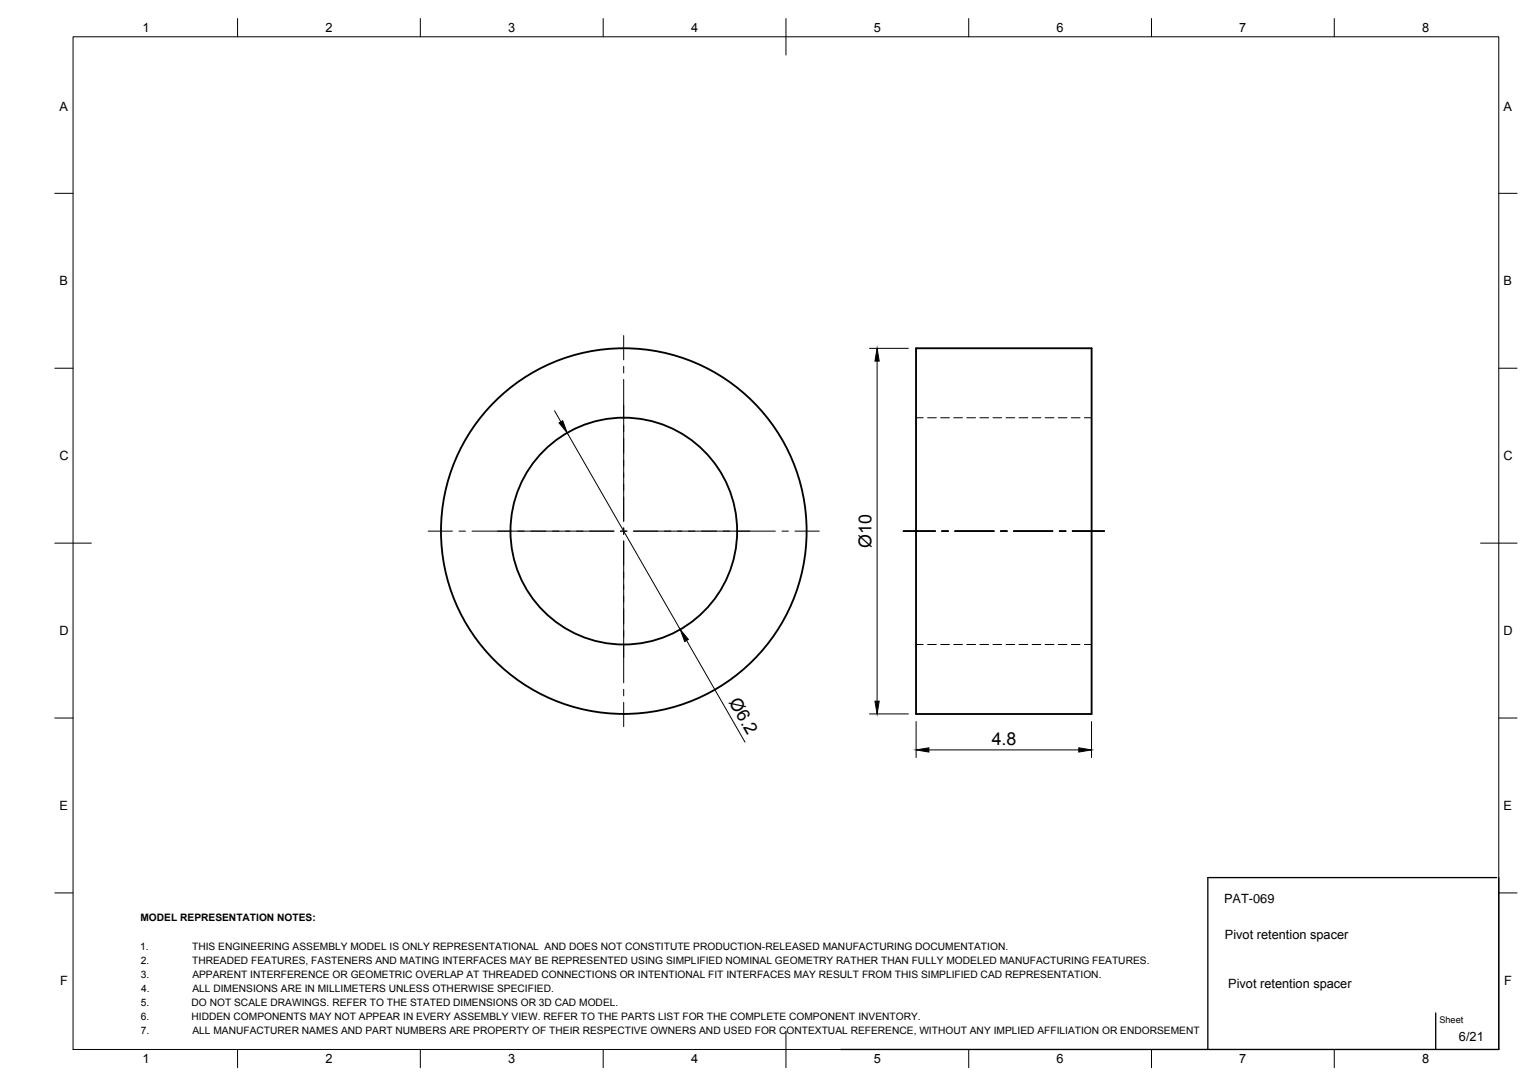
ISO-10303-21;
HEADER;
/* Generated by software containing ST-Developer
 * from STEP Tools, Inc. (www.steptools.com) 
 */

FILE_DESCRIPTION(
/* description */ ('Located fixture plate with toggle clamp'),
/* implementation_level */ '2;1');

FILE_NAME(
/* name */ 'Pivot retention spacer.step',
/* time_stamp */ '2026-10-27T21:36:12-07:00',
/* author */ (''),
/* organization */ (''),
/* preprocessor_version */ 'ST-DEVELOPER v20.2',
/* originating_system */ 'Autodesk Translation Framework v15.17.0.0',
/* authorisation */ '');

FILE_SCHEMA (('AUTOMOTIVE_DESIGN { 1 0 10303 214 3 1 1 }'));
ENDSEC;

DATA;
#10=MECHANICAL_DESIGN_GEOMETRIC_PRESENTATION_REPRESENTATION('',(#343),#9285);
#295=SHAPE_REPRESENTATION_RELATIONSHIP('SRR','None',#9421,#319);
#319=ADVANCED_BREP_SHAPE_REPRESENTATION('',(#364),#9283);
#343=STYLED_ITEM('',(#9626),#364);
#364=MANIFOLD_SOLID_BREP('Body1',#5194);
#483=FACE_BOUND('',#1374,.T.);
#484=FACE_BOUND('',#1376,.T.);
#668=PLANE('',#5971);
#669=PLANE('',#5972);
#959=FACE_OUTER_BOUND('',#1371,.T.);
#960=FACE_OUTER_BOUND('',#1372,.T.);
#961=FACE_OUTER_BOUND('',#1373,.T.);
#962=FACE_OUTER_BOUND('',#1375,.T.);
#1371=EDGE_LOOP('',(#4756,#4757,#4758,#4759));
#1372=EDGE_LOOP('',(#4760,#4761,#4762,#4763));
#1373=EDGE_LOOP('',(#4764));
#1374=EDGE_LOOP('',(#4765));
#1375=EDGE_LOOP('',(#4766));
#1376=EDGE_LOOP('',(#4767));
#1572=CIRCLE('',#5966,0.31);
#1573=CIRCLE('',#5967,0.31);
#1574=CIRCLE('',#5969,0.5);
#1575=CIRCLE('',#5970,0.5);
#1984=LINE('',#9095,#2394);
#1985=LINE('',#9101,#2395);
#2394=VECTOR('',#7444,0.31);
#2395=VECTOR('',#7451,0.5);
#2818=VERTEX_POINT('',#9092);
#2819=VERTEX_POINT('',#9094);
#2820=VERTEX_POINT('',#9098);
#2821=VERTEX_POINT('',#9100);
#3466=EDGE_CURVE('',#2818,#2818,#1572,.T.);
#3467=EDGE_CURVE('',#2818,#2819,#1984,.T.);
#3468=EDGE_CURVE('',#2819,#2819,#1573,.T.);
#3469=EDGE_CURVE('',#2820,#2820,#1574,.T.);
#3470=EDGE_CURVE('',#2820,#2821,#1985,.T.);
#3471=EDGE_CURVE('',#2821,#2821,#1575,.T.);
#4756=ORIENTED_EDGE('',*,*,#3466,.F.);
#4757=ORIENTED_EDGE('',*,*,#3467,.T.);
#4758=ORIENTED_EDGE('',*,*,#3468,.T.);
#4759=ORIENTED_EDGE('',*,*,#3467,.F.);
#4760=ORIENTED_EDGE('',*,*,#3469,.F.);
#4761=ORIENTED_EDGE('',*,*,#3470,.T.);
#4762=ORIENTED_EDGE('',*,*,#3471,.T.);
#4763=ORIENTED_EDGE('',*,*,#3470,.F.);
#4764=ORIENTED_EDGE('',*,*,#3469,.T.);
#4765=ORIENTED_EDGE('',*,*,#3466,.T.);
#4766=ORIENTED_EDGE('',*,*,#3471,.F.);
#4767=ORIENTED_EDGE('',*,*,#3468,.F.);
#4871=CYLINDRICAL_SURFACE('',#5965,0.31);
#4872=CYLINDRICAL_SURFACE('',#5968,0.5);
#5160=ADVANCED_FACE('',(#959),#4871,.F.);
#5161=ADVANCED_FACE('',(#960),#4872,.T.);
#5162=ADVANCED_FACE('',(#961,#483),#668,.T.);
#5163=ADVANCED_FACE('',(#962,#484),#669,.F.);
#5194=CLOSED_SHELL('',(#5160,#5161,#5162,#5163));
#5964=AXIS2_PLACEMENT_3D('',#9090,#7438,#7439);
#5965=AXIS2_PLACEMENT_3D('',#9091,#7440,#7441);
#5966=AXIS2_PLACEMENT_3D('',#9093,#7442,#7443);
#5967=AXIS2_PLACEMENT_3D('',#9096,#7445,#7446);
#5968=AXIS2_PLACEMENT_3D('',#9097,#7447,#7448);
#5969=AXIS2_PLACEMENT_3D('',#9099,#7449,#7450);
#5970=AXIS2_PLACEMENT_3D('',#9102,#7452,#7453);
#5971=AXIS2_PLACEMENT_3D('',#9103,#7454,#7455);
#5972=AXIS2_PLACEMENT_3D('',#9104,#7456,#7457);
#7438=DIRECTION('axis',(0.,0.,1.));
#7439=DIRECTION('refdir',(1.,0.,0.));
#7440=DIRECTION('center_axis',(0.,1.,0.));
#7441=DIRECTION('ref_axis',(1.,0.,0.));
#7442=DIRECTION('center_axis',(0.,-1.,0.));
#7443=DIRECTION('ref_axis',(1.,0.,0.));
#7444=DIRECTION('',(0.,-1.,0.));
#7445=DIRECTION('center_axis',(0.,-1.,0.));
#7446=DIRECTION('ref_axis',(1.,0.,0.));
#7447=DIRECTION('center_axis',(0.,1.,0.));
#7448=DIRECTION('ref_axis',(1.,0.,0.));
#7449=DIRECTION('center_axis',(0.,1.,0.));
#7450=DIRECTION('ref_axis',(1.,0.,0.));
#7451=DIRECTION('',(0.,-1.,0.));
#7452=DIRECTION('center_axis',(0.,1.,0.));
#7453=DIRECTION('ref_axis',(1.,0.,0.));
#7454=DIRECTION('center_axis',(0.,1.,0.));
#7455=DIRECTION('ref_axis',(1.,0.,0.));
#7456=DIRECTION('center_axis',(0.,1.,0.));
#7457=DIRECTION('ref_axis',(1.,0.,0.));
#9090=CARTESIAN_POINT('',(0.,0.,0.));
#9091=CARTESIAN_POINT('Origin',(0.,-1.54,2.5));
#9092=CARTESIAN_POINT('',(-0.31,-1.06,2.5));
#9093=CARTESIAN_POINT('Origin',(0.,-1.06,2.5));
#9094=CARTESIAN_POINT('',(-0.31,-1.54,2.5));
#9095=CARTESIAN_POINT('',(-0.31,-1.54,2.5));
#9096=CARTESIAN_POINT('Origin',(0.,-1.54,2.5));
#9097=CARTESIAN_POINT('Origin',(0.,-1.54,2.5));
#9098=CARTESIAN_POINT('',(-0.5,-1.06,2.5));
#9099=CARTESIAN_POINT('Origin',(0.,-1.06,2.5));
#9100=CARTESIAN_POINT('',(-0.5,-1.54,2.5));
#9101=CARTESIAN_POINT('',(-0.5,-1.54,2.5));
#9102=CARTESIAN_POINT('Origin',(0.,-1.54,2.5));
#9103=CARTESIAN_POINT('Origin',(0.,-1.06,2.5));
#9104=CARTESIAN_POINT('Origin',(0.,-1.54,2.5));
#9253=UNCERTAINTY_MEASURE_WITH_UNIT(LENGTH_MEASURE(0.001),#9286,
'DISTANCE_ACCURACY_VALUE',
'Maximum model space distance between geometric entities at asserted c
onnectivities');
#9255=UNCERTAINTY_MEASURE_WITH_UNIT(LENGTH_MEASURE(0.001),#9286,
'DISTANCE_ACCURACY_VALUE',
'Maximum model space distance between geometric entities at asserted c
onnectivities');
#9283=(
GEOMETRIC_REPRESENTATION_CONTEXT(3)
GLOBAL_UNCERTAINTY_ASSIGNED_CONTEXT((#9253))
GLOBAL_UNIT_ASSIGNED_CONTEXT((#9286,#9288,#9289))
REPRESENTATION_CONTEXT('','3D')
);
#9285=(
GEOMETRIC_REPRESENTATION_CONTEXT(3)
GLOBAL_UNCERTAINTY_ASSIGNED_CONTEXT((#9255))
GLOBAL_UNIT_ASSIGNED_CONTEXT((#9286,#9288,#9289))
REPRESENTATION_CONTEXT('','3D')
);
#9286=(
LENGTH_UNIT()
NAMED_UNIT(*)
SI_UNIT(.CENTI.,.METRE.)
);
#9288=(
NAMED_UNIT(*)
PLANE_ANGLE_UNIT()
SI_UNIT($,.RADIAN.)
);
#9289=(
NAMED_UNIT(*)
SI_UNIT($,.STERADIAN.)
SOLID_ANGLE_UNIT()
);
#9317=SHAPE_DEFINITION_REPRESENTATION(#9347,#9421);
#9347=PRODUCT_DEFINITION_SHAPE('',$,#9451);
#9421=SHAPE_REPRESENTATION('',(#5964),#9283);
#9423=PRODUCT_DEFINITION_CONTEXT('part definition',#9512,'design');
#9451=PRODUCT_DEFINITION('Pivot retention spacer',
'Pivot retention spacer',#9480,#9423);
#9480=PRODUCT_DEFINITION_FORMATION('',$,#9541);
#9512=APPLICATION_CONTEXT(
'Core Data for Automotive Mechanical Design Process');
#9513=PRODUCT_CONTEXT('part definition',#9512,'mechanical');
#9541=PRODUCT('Pivot retention spacer','Pivot retention spacer',
'Pivot retention spacer',(#9513));
#9620=COLOUR_RGB('Off White',0.89,0.88,0.83);
#9621=FILL_AREA_STYLE_COLOUR('',#9620);
#9622=FILL_AREA_STYLE('',(#9621));
#9623=SURFACE_STYLE_FILL_AREA(#9622);
#9624=SURFACE_SIDE_STYLE('',(#9623));
#9625=SURFACE_STYLE_USAGE(.BOTH.,#9624);
#9626=PRESENTATION_STYLE_ASSIGNMENT((#9625));
ENDSEC;
END-ISO-10303-21;
